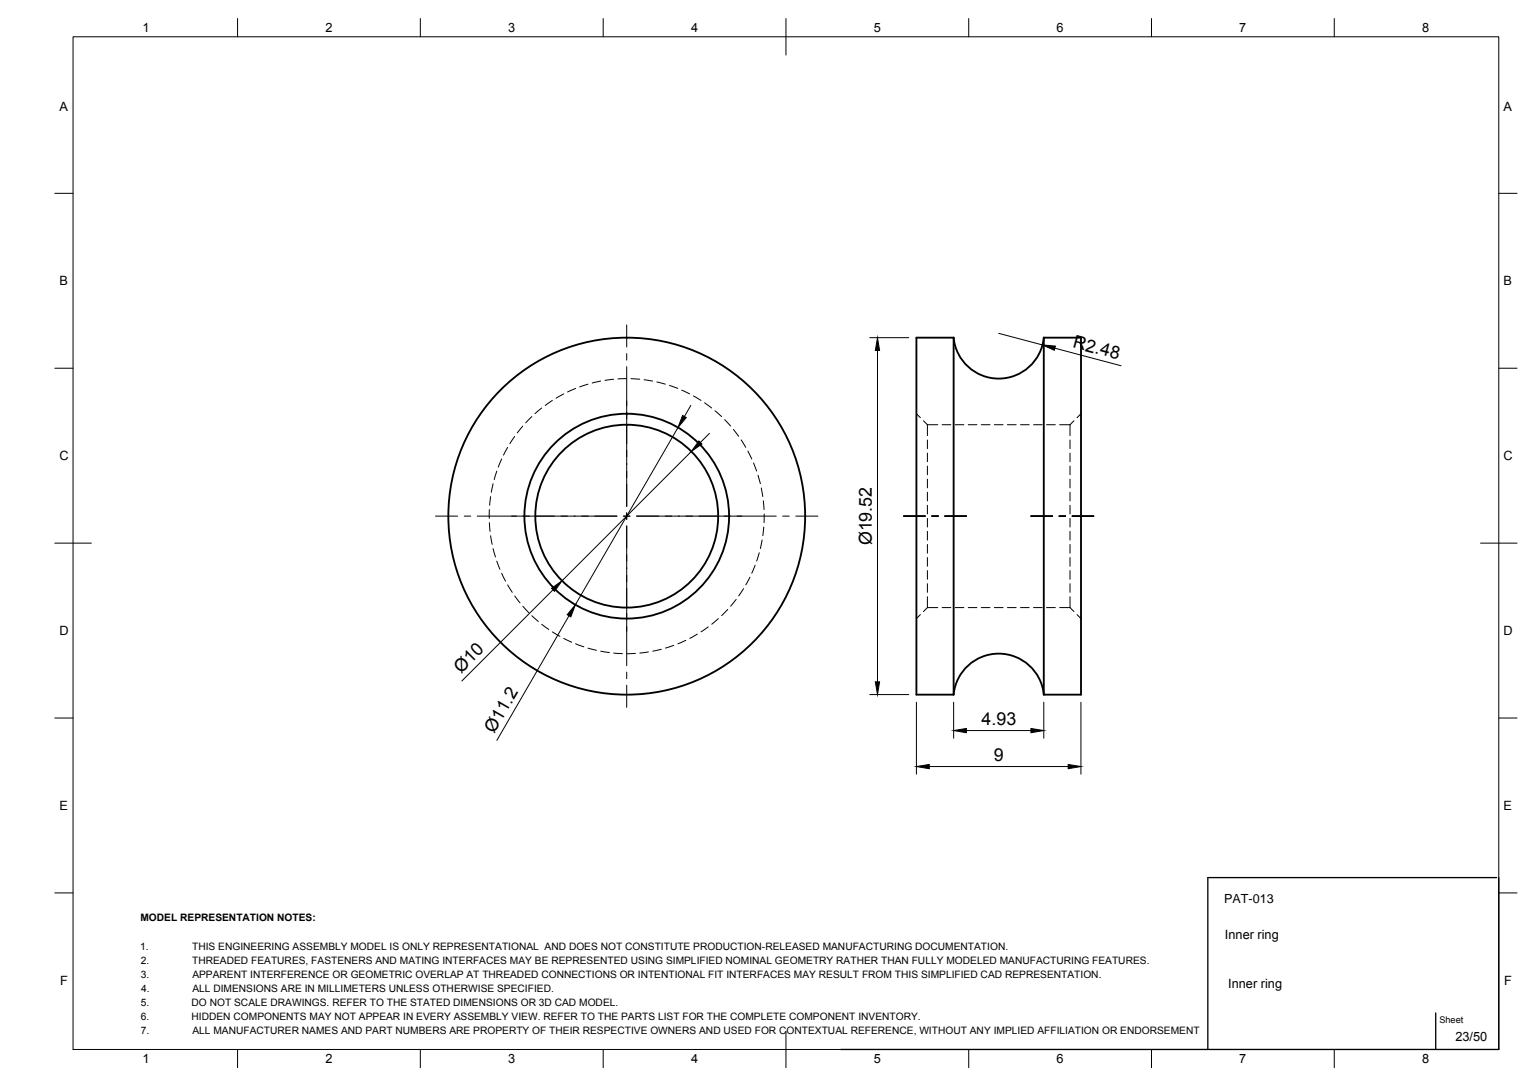
ISO-10303-21;
HEADER;
/* Generated by software containing ST-Developer
 * from STEP Tools, Inc. (www.steptools.com) 
 */

FILE_DESCRIPTION(
/* description */ ('Belt-driven linear axis on 2020 extrusion'),
/* implementation_level */ '2;1');

FILE_NAME(
/* name */ 'Inner ring.step',
/* time_stamp */ '2026-10-28T03:26:09-07:00',
/* author */ (''),
/* organization */ (''),
/* preprocessor_version */ 'ST-DEVELOPER v20.2',
/* originating_system */ 'Autodesk Translation Framework v15.17.0.0',
/* authorisation */ '');

FILE_SCHEMA (('AUTOMOTIVE_DESIGN { 1 0 10303 214 3 1 1 }'));
ENDSEC;

DATA;
#10=MECHANICAL_DESIGN_GEOMETRIC_PRESENTATION_REPRESENTATION('',(#626),#20096);
#497=CONICAL_SURFACE('',#11929,0.53,0.785398163397448);
#498=CONICAL_SURFACE('',#11936,0.53,0.785398163397448);
#516=TOROIDAL_SURFACE('',#11918,1.,0.247676);
#532=SHAPE_REPRESENTATION_RELATIONSHIP('SRR','None',#20329,#578);
#578=ADVANCED_BREP_SHAPE_REPRESENTATION('',(#682),#20060);
#626=STYLED_ITEM('',(#20650),#682);
#682=MANIFOLD_SOLID_BREP('Body1',#10939);
#804=FACE_BOUND('',#2177,.T.);
#805=FACE_BOUND('',#2180,.T.);
#1005=PLANE('',#11931);
#1006=PLANE('',#11934);
#1464=FACE_OUTER_BOUND('',#2172,.T.);
#1465=FACE_OUTER_BOUND('',#2173,.T.);
#1466=FACE_OUTER_BOUND('',#2174,.T.);
#1467=FACE_OUTER_BOUND('',#2175,.T.);
#1468=FACE_OUTER_BOUND('',#2176,.T.);
#1469=FACE_OUTER_BOUND('',#2178,.T.);
#1470=FACE_OUTER_BOUND('',#2179,.T.);
#1471=FACE_OUTER_BOUND('',#2181,.T.);
#2172=EDGE_LOOP('',(#8225,#8226,#8227,#8228,#8229,#8230));
#2173=EDGE_LOOP('',(#8231,#8232,#8233,#8234,#8235));
#2174=EDGE_LOOP('',(#8236,#8237,#8238,#8239));
#2175=EDGE_LOOP('',(#8240,#8241,#8242,#8243));
#2176=EDGE_LOOP('',(#8244));
#2177=EDGE_LOOP('',(#8245));
#2178=EDGE_LOOP('',(#8246,#8247,#8248,#8249,#8250));
#2179=EDGE_LOOP('',(#8251));
#2180=EDGE_LOOP('',(#8252));
#2181=EDGE_LOOP('',(#8253,#8254,#8255,#8256));
#2955=LINE('',#17286,#3812);
#2956=LINE('',#17292,#3813);
#2957=LINE('',#17296,#3814);
#2958=LINE('',#17302,#3815);
#2959=LINE('',#17307,#3816);
#3812=VECTOR('',#13945,0.976185);
#3813=VECTOR('',#13952,0.5);
#3814=VECTOR('',#13957,0.53);
#3815=VECTOR('',#13966,0.976185);
#3816=VECTOR('',#13973,0.53);
#4575=CIRCLE('',#11919,0.976185);
#4576=CIRCLE('',#11920,0.976185);
#4577=CIRCLE('',#11921,0.247676);
#4578=CIRCLE('',#11922,0.976185);
#4579=CIRCLE('',#11923,0.976185);
#4580=CIRCLE('',#11925,0.976185);
#4581=CIRCLE('',#11927,0.5);
#4582=CIRCLE('',#11928,0.5);
#4583=CIRCLE('',#11930,0.56);
#4584=CIRCLE('',#11933,0.976185);
#4585=CIRCLE('',#11935,0.56);
#5216=VERTEX_POINT('',#17275);
#5217=VERTEX_POINT('',#17276);
#5218=VERTEX_POINT('',#17279);
#5219=VERTEX_POINT('',#17281);
#5220=VERTEX_POINT('',#17285);
#5221=VERTEX_POINT('',#17289);
#5222=VERTEX_POINT('',#17291);
#5223=VERTEX_POINT('',#17295);
#5224=VERTEX_POINT('',#17300);
#5225=VERTEX_POINT('',#17304);
#6327=EDGE_CURVE('',#5216,#5217,#4575,.T.);
#6328=EDGE_CURVE('',#5217,#5216,#4576,.T.);
#6329=EDGE_CURVE('',#5217,#5218,#4577,.T.);
#6330=EDGE_CURVE('',#5219,#5218,#4578,.T.);
#6331=EDGE_CURVE('',#5218,#5219,#4579,.T.);
#6332=EDGE_CURVE('',#5219,#5220,#2955,.T.);
#6333=EDGE_CURVE('',#5220,#5220,#4580,.T.);
#6334=EDGE_CURVE('',#5221,#5221,#4581,.T.);
#6335=EDGE_CURVE('',#5221,#5222,#2956,.T.);
#6336=EDGE_CURVE('',#5222,#5222,#4582,.T.);
#6337=EDGE_CURVE('',#5222,#5223,#2957,.T.);
#6338=EDGE_CURVE('',#5223,#5223,#4583,.T.);
#6339=EDGE_CURVE('',#5224,#5224,#4584,.T.);
#6340=EDGE_CURVE('',#5224,#5216,#2958,.T.);
#6341=EDGE_CURVE('',#5225,#5225,#4585,.T.);
#6342=EDGE_CURVE('',#5225,#5221,#2959,.T.);
#8225=ORIENTED_EDGE('',*,*,#6327,.F.);
#8226=ORIENTED_EDGE('',*,*,#6328,.F.);
#8227=ORIENTED_EDGE('',*,*,#6329,.T.);
#8228=ORIENTED_EDGE('',*,*,#6330,.F.);
#8229=ORIENTED_EDGE('',*,*,#6331,.F.);
#8230=ORIENTED_EDGE('',*,*,#6329,.F.);
#8231=ORIENTED_EDGE('',*,*,#6330,.T.);
#8232=ORIENTED_EDGE('',*,*,#6331,.T.);
#8233=ORIENTED_EDGE('',*,*,#6332,.T.);
#8234=ORIENTED_EDGE('',*,*,#6333,.T.);
#8235=ORIENTED_EDGE('',*,*,#6332,.F.);
#8236=ORIENTED_EDGE('',*,*,#6334,.T.);
#8237=ORIENTED_EDGE('',*,*,#6335,.T.);
#8238=ORIENTED_EDGE('',*,*,#6336,.F.);
#8239=ORIENTED_EDGE('',*,*,#6335,.F.);
#8240=ORIENTED_EDGE('',*,*,#6336,.T.);
#8241=ORIENTED_EDGE('',*,*,#6337,.T.);
#8242=ORIENTED_EDGE('',*,*,#6338,.F.);
#8243=ORIENTED_EDGE('',*,*,#6337,.F.);
#8244=ORIENTED_EDGE('',*,*,#6333,.F.);
#8245=ORIENTED_EDGE('',*,*,#6338,.T.);
#8246=ORIENTED_EDGE('',*,*,#6339,.F.);
#8247=ORIENTED_EDGE('',*,*,#6340,.T.);
#8248=ORIENTED_EDGE('',*,*,#6327,.T.);
#8249=ORIENTED_EDGE('',*,*,#6328,.T.);
#8250=ORIENTED_EDGE('',*,*,#6340,.F.);
#8251=ORIENTED_EDGE('',*,*,#6339,.T.);
#8252=ORIENTED_EDGE('',*,*,#6341,.F.);
#8253=ORIENTED_EDGE('',*,*,#6341,.T.);
#8254=ORIENTED_EDGE('',*,*,#6342,.T.);
#8255=ORIENTED_EDGE('',*,*,#6334,.F.);
#8256=ORIENTED_EDGE('',*,*,#6342,.F.);
#10175=CYLINDRICAL_SURFACE('',#11924,0.976185);
#10176=CYLINDRICAL_SURFACE('',#11926,0.5);
#10177=CYLINDRICAL_SURFACE('',#11932,0.976185);
#10515=ADVANCED_FACE('',(#1464),#516,.F.);
#10516=ADVANCED_FACE('',(#1465),#10175,.T.);
#10517=ADVANCED_FACE('',(#1466),#10176,.F.);
#10518=ADVANCED_FACE('',(#1467),#497,.F.);
#10519=ADVANCED_FACE('',(#1468,#804),#1005,.T.);
#10520=ADVANCED_FACE('',(#1469),#10177,.T.);
#10521=ADVANCED_FACE('',(#1470,#805),#1006,.T.);
#10522=ADVANCED_FACE('',(#1471),#498,.F.);
#10939=CLOSED_SHELL('',(#10515,#10516,#10517,#10518,#10519,#10520,#10521,
#10522));
#11917=AXIS2_PLACEMENT_3D('',#17273,#13929,#13930);
#11918=AXIS2_PLACEMENT_3D('',#17274,#13931,#13932);
#11919=AXIS2_PLACEMENT_3D('',#17277,#13933,#13934);
#11920=AXIS2_PLACEMENT_3D('',#17278,#13935,#13936);
#11921=AXIS2_PLACEMENT_3D('',#17280,#13937,#13938);
#11922=AXIS2_PLACEMENT_3D('',#17282,#13939,#13940);
#11923=AXIS2_PLACEMENT_3D('',#17283,#13941,#13942);
#11924=AXIS2_PLACEMENT_3D('',#17284,#13943,#13944);
#11925=AXIS2_PLACEMENT_3D('',#17287,#13946,#13947);
#11926=AXIS2_PLACEMENT_3D('',#17288,#13948,#13949);
#11927=AXIS2_PLACEMENT_3D('',#17290,#13950,#13951);
#11928=AXIS2_PLACEMENT_3D('',#17293,#13953,#13954);
#11929=AXIS2_PLACEMENT_3D('',#17294,#13955,#13956);
#11930=AXIS2_PLACEMENT_3D('',#17297,#13958,#13959);
#11931=AXIS2_PLACEMENT_3D('',#17298,#13960,#13961);
#11932=AXIS2_PLACEMENT_3D('',#17299,#13962,#13963);
#11933=AXIS2_PLACEMENT_3D('',#17301,#13964,#13965);
#11934=AXIS2_PLACEMENT_3D('',#17303,#13967,#13968);
#11935=AXIS2_PLACEMENT_3D('',#17305,#13969,#13970);
#11936=AXIS2_PLACEMENT_3D('',#17306,#13971,#13972);
#13929=DIRECTION('axis',(0.,0.,1.));
#13930=DIRECTION('refdir',(1.,0.,0.));
#13931=DIRECTION('center_axis',(0.,-1.,0.));
#13932=DIRECTION('ref_axis',(0.,0.,-1.));
#13933=DIRECTION('center_axis',(0.,-1.,0.));
#13934=DIRECTION('ref_axis',(1.,0.,0.));
#13935=DIRECTION('center_axis',(0.,-1.,0.));
#13936=DIRECTION('ref_axis',(1.,0.,0.));
#13937=DIRECTION('center_axis',(1.,0.,1.22464679914735E-16));
#13938=DIRECTION('ref_axis',(-1.22464679914735E-16,0.,1.));
#13939=DIRECTION('center_axis',(0.,1.,0.));
#13940=DIRECTION('ref_axis',(1.,0.,0.));
#13941=DIRECTION('center_axis',(0.,1.,0.));
#13942=DIRECTION('ref_axis',(1.,0.,0.));
#13943=DIRECTION('center_axis',(0.,-1.,0.));
#13944=DIRECTION('ref_axis',(1.,0.,0.));
#13945=DIRECTION('',(0.,1.,0.));
#13946=DIRECTION('center_axis',(0.,-1.,0.));
#13947=DIRECTION('ref_axis',(1.,0.,0.));
#13948=DIRECTION('center_axis',(0.,-1.,0.));
#13949=DIRECTION('ref_axis',(1.,0.,0.));
#13950=DIRECTION('center_axis',(0.,-1.,0.));
#13951=DIRECTION('ref_axis',(1.,0.,0.));
#13952=DIRECTION('',(0.,1.,0.));
#13953=DIRECTION('center_axis',(0.,-1.,0.));
#13954=DIRECTION('ref_axis',(1.,0.,0.));
#13955=DIRECTION('center_axis',(0.,1.,0.));
#13956=DIRECTION('ref_axis',(1.,0.,0.));
#13957=DIRECTION('',(-0.707106781186547,0.707106781186548,-8.65956056235493E-17));
#13958=DIRECTION('center_axis',(0.,-1.,0.));
#13959=DIRECTION('ref_axis',(1.,0.,0.));
#13960=DIRECTION('center_axis',(0.,1.,0.));
#13961=DIRECTION('ref_axis',(0.,0.,1.));
#13962=DIRECTION('center_axis',(0.,-1.,0.));
#13963=DIRECTION('ref_axis',(1.,0.,0.));
#13964=DIRECTION('center_axis',(0.,-1.,0.));
#13965=DIRECTION('ref_axis',(1.,0.,0.));
#13966=DIRECTION('',(0.,1.,0.));
#13967=DIRECTION('center_axis',(0.,-1.,0.));
#13968=DIRECTION('ref_axis',(0.,0.,-1.));
#13969=DIRECTION('center_axis',(0.,-1.,0.));
#13970=DIRECTION('ref_axis',(1.,0.,0.));
#13971=DIRECTION('center_axis',(0.,-1.,0.));
#13972=DIRECTION('ref_axis',(1.,0.,0.));
#13973=DIRECTION('',(0.707106781186547,0.707106781186548,8.65956056235493E-17));
#17273=CARTESIAN_POINT('',(0.,0.,0.));
#17274=CARTESIAN_POINT('Origin',(0.,0.,0.));
#17275=CARTESIAN_POINT('',(-0.976185,-0.246528389340863,-1.19548183562566E-16));
#17276=CARTESIAN_POINT('',(-1.19548183562566E-16,-0.246528389340863,0.976185));
#17277=CARTESIAN_POINT('Origin',(0.,-0.246528389340863,0.));
#17278=CARTESIAN_POINT('Origin',(0.,-0.246528389340863,0.));
#17279=CARTESIAN_POINT('',(-1.19548183562566E-16,0.246528389340863,0.976185));
#17280=CARTESIAN_POINT('Origin',(-1.22464679914735E-16,0.,1.));
#17281=CARTESIAN_POINT('',(-0.976185,0.246528389340863,1.19548183562566E-16));
#17282=CARTESIAN_POINT('Origin',(0.,0.246528389340863,0.));
#17283=CARTESIAN_POINT('Origin',(0.,0.246528389340863,0.));
#17284=CARTESIAN_POINT('Origin',(0.,0.,0.));
#17285=CARTESIAN_POINT('',(-0.976185,0.45,-1.19548183562566E-16));
#17286=CARTESIAN_POINT('',(-0.976185,0.,-1.19548183562566E-16));
#17287=CARTESIAN_POINT('Origin',(0.,0.45,0.));
#17288=CARTESIAN_POINT('Origin',(0.,0.,0.));
#17289=CARTESIAN_POINT('',(-0.5,-0.39,-6.12323399573677E-17));
#17290=CARTESIAN_POINT('Origin',(0.,-0.39,0.));
#17291=CARTESIAN_POINT('',(-0.5,0.39,-6.12323399573677E-17));
#17292=CARTESIAN_POINT('',(-0.5,0.,-6.12323399573677E-17));
#17293=CARTESIAN_POINT('Origin',(0.,0.39,0.));
#17294=CARTESIAN_POINT('Origin',(0.,0.42,0.));
#17295=CARTESIAN_POINT('',(-0.56,0.45,-6.85802207522518E-17));
#17296=CARTESIAN_POINT('',(-0.53,0.42,-6.49062803548097E-17));
#17297=CARTESIAN_POINT('Origin',(0.,0.45,0.));
#17298=CARTESIAN_POINT('Origin',(0.976185,0.45,0.));
#17299=CARTESIAN_POINT('Origin',(0.,0.,0.));
#17300=CARTESIAN_POINT('',(-0.976185,-0.45,-1.19548183562566E-16));
#17301=CARTESIAN_POINT('Origin',(0.,-0.45,0.));
#17302=CARTESIAN_POINT('',(-0.976185,0.,-1.19548183562566E-16));
#17303=CARTESIAN_POINT('Origin',(0.56,-0.45,0.));
#17304=CARTESIAN_POINT('',(-0.56,-0.45,-6.85802207522518E-17));
#17305=CARTESIAN_POINT('Origin',(0.,-0.45,0.));
#17306=CARTESIAN_POINT('Origin',(0.,-0.42,0.));
#17307=CARTESIAN_POINT('',(-0.53,-0.42,-6.49062803548097E-17));
#20006=UNCERTAINTY_MEASURE_WITH_UNIT(LENGTH_MEASURE(0.001),#20097,
'DISTANCE_ACCURACY_VALUE',
'Maximum model space distance between geometric entities at asserted c
onnectivities');
#20042=UNCERTAINTY_MEASURE_WITH_UNIT(LENGTH_MEASURE(0.001),#20097,
'DISTANCE_ACCURACY_VALUE',
'Maximum model space distance between geometric entities at asserted c
onnectivities');
#20060=(
GEOMETRIC_REPRESENTATION_CONTEXT(3)
GLOBAL_UNCERTAINTY_ASSIGNED_CONTEXT((#20006))
GLOBAL_UNIT_ASSIGNED_CONTEXT((#20097,#20099,#20100))
REPRESENTATION_CONTEXT('','3D')
);
#20096=(
GEOMETRIC_REPRESENTATION_CONTEXT(3)
GLOBAL_UNCERTAINTY_ASSIGNED_CONTEXT((#20042))
GLOBAL_UNIT_ASSIGNED_CONTEXT((#20097,#20099,#20100))
REPRESENTATION_CONTEXT('','3D')
);
#20097=(
LENGTH_UNIT()
NAMED_UNIT(*)
SI_UNIT(.CENTI.,.METRE.)
);
#20099=(
NAMED_UNIT(*)
PLANE_ANGLE_UNIT()
SI_UNIT($,.RADIAN.)
);
#20100=(
NAMED_UNIT(*)
SI_UNIT($,.STERADIAN.)
SOLID_ANGLE_UNIT()
);
#20118=SHAPE_DEFINITION_REPRESENTATION(#20171,#20329);
#20171=PRODUCT_DEFINITION_SHAPE('',$,#20383);
#20329=SHAPE_REPRESENTATION('',(#11917),#20060);
#20365=PRODUCT_DEFINITION_CONTEXT('part definition',#20526,'design');
#20383=PRODUCT_DEFINITION('Inner ring','Inner ring',#20436,#20365);
#20436=PRODUCT_DEFINITION_FORMATION('',$,#20545);
#20526=APPLICATION_CONTEXT(
'Core Data for Automotive Mechanical Design Process');
#20527=PRODUCT_CONTEXT('part definition',#20526,'mechanical');
#20545=PRODUCT('Inner ring','Inner ring','Inner ring',(#20527));
#20644=COLOUR_RGB('Grey',0.48,0.52,0.57);
#20645=FILL_AREA_STYLE_COLOUR('',#20644);
#20646=FILL_AREA_STYLE('',(#20645));
#20647=SURFACE_STYLE_FILL_AREA(#20646);
#20648=SURFACE_SIDE_STYLE('',(#20647));
#20649=SURFACE_STYLE_USAGE(.BOTH.,#20648);
#20650=PRESENTATION_STYLE_ASSIGNMENT((#20649));
ENDSEC;
END-ISO-10303-21;
